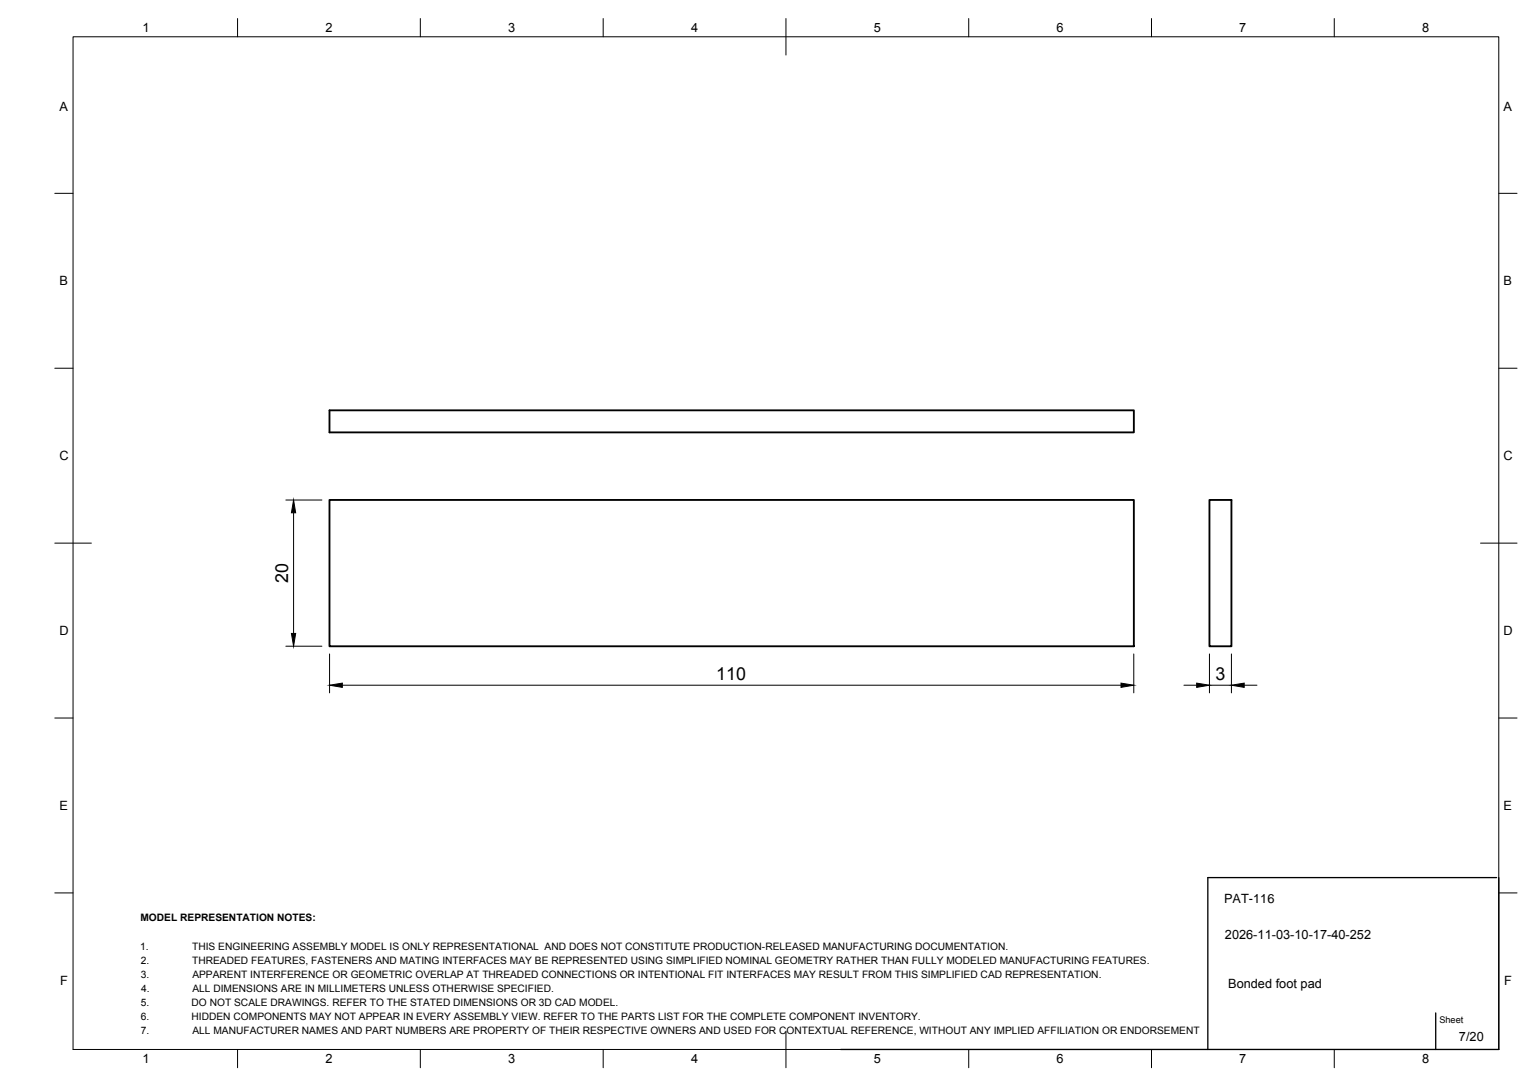
ISO-10303-21;
HEADER;
/* Generated by software containing ST-Developer
 * from STEP Tools, Inc. (www.steptools.com) 
 */

FILE_DESCRIPTION(
/* description */ ('V-block with clamp strap'),
/* implementation_level */ '2;1');

FILE_NAME(
/* name */ 'Bonded foot pad.step',
/* time_stamp */ '2026-10-27T10:50:53-07:00',
/* author */ (''),
/* organization */ (''),
/* preprocessor_version */ 'ST-DEVELOPER v20.2',
/* originating_system */ 'Autodesk Translation Framework v15.17.0.0',
/* authorisation */ '');

FILE_SCHEMA (('AUTOMOTIVE_DESIGN { 1 0 10303 214 3 1 1 }'));
ENDSEC;

DATA;
#10=MECHANICAL_DESIGN_GEOMETRIC_PRESENTATION_REPRESENTATION('',(#268),#7344);
#226=SHAPE_REPRESENTATION_RELATIONSHIP('SRR','None',#7444,#247);
#247=ADVANCED_BREP_SHAPE_REPRESENTATION('',(#289),#7323);
#268=STYLED_ITEM('',(#7624),#289);
#289=MANIFOLD_SOLID_BREP('Body1',#4150);
#598=FACE_OUTER_BOUND('',#868,.T.);
#599=FACE_OUTER_BOUND('',#869,.T.);
#600=FACE_OUTER_BOUND('',#870,.T.);
#601=FACE_OUTER_BOUND('',#871,.T.);
#602=FACE_OUTER_BOUND('',#872,.T.);
#603=FACE_OUTER_BOUND('',#873,.T.);
#868=EDGE_LOOP('',(#2876,#2877,#2878,#2879));
#869=EDGE_LOOP('',(#2880,#2881,#2882,#2883));
#870=EDGE_LOOP('',(#2884,#2885,#2886,#2887));
#871=EDGE_LOOP('',(#2888,#2889,#2890,#2891));
#872=EDGE_LOOP('',(#2892,#2893,#2894,#2895));
#873=EDGE_LOOP('',(#2896,#2897,#2898,#2899));
#1175=LINE('',#6280,#1540);
#1176=LINE('',#6282,#1541);
#1177=LINE('',#6284,#1542);
#1178=LINE('',#6285,#1543);
#1179=LINE('',#6288,#1544);
#1180=LINE('',#6290,#1545);
#1181=LINE('',#6291,#1546);
#1182=LINE('',#6294,#1547);
#1183=LINE('',#6296,#1548);
#1184=LINE('',#6297,#1549);
#1185=LINE('',#6299,#1550);
#1186=LINE('',#6300,#1551);
#1540=VECTOR('',#5045,1.);
#1541=VECTOR('',#5046,1.);
#1542=VECTOR('',#5047,1.);
#1543=VECTOR('',#5048,1.);
#1544=VECTOR('',#5051,1.);
#1545=VECTOR('',#5052,1.);
#1546=VECTOR('',#5053,1.);
#1547=VECTOR('',#5056,1.);
#1548=VECTOR('',#5057,1.);
#1549=VECTOR('',#5058,1.);
#1550=VECTOR('',#5061,1.);
#1551=VECTOR('',#5062,1.);
#1903=VERTEX_POINT('',#6278);
#1904=VERTEX_POINT('',#6279);
#1905=VERTEX_POINT('',#6281);
#1906=VERTEX_POINT('',#6283);
#1907=VERTEX_POINT('',#6287);
#1908=VERTEX_POINT('',#6289);
#1909=VERTEX_POINT('',#6293);
#1910=VERTEX_POINT('',#6295);
#2264=EDGE_CURVE('',#1903,#1904,#1175,.T.);
#2265=EDGE_CURVE('',#1904,#1905,#1176,.T.);
#2266=EDGE_CURVE('',#1906,#1905,#1177,.T.);
#2267=EDGE_CURVE('',#1903,#1906,#1178,.T.);
#2268=EDGE_CURVE('',#1907,#1903,#1179,.T.);
#2269=EDGE_CURVE('',#1908,#1906,#1180,.T.);
#2270=EDGE_CURVE('',#1907,#1908,#1181,.T.);
#2271=EDGE_CURVE('',#1909,#1907,#1182,.T.);
#2272=EDGE_CURVE('',#1910,#1908,#1183,.T.);
#2273=EDGE_CURVE('',#1909,#1910,#1184,.T.);
#2274=EDGE_CURVE('',#1904,#1909,#1185,.T.);
#2275=EDGE_CURVE('',#1905,#1910,#1186,.T.);
#2876=ORIENTED_EDGE('',*,*,#2264,.T.);
#2877=ORIENTED_EDGE('',*,*,#2265,.T.);
#2878=ORIENTED_EDGE('',*,*,#2266,.F.);
#2879=ORIENTED_EDGE('',*,*,#2267,.F.);
#2880=ORIENTED_EDGE('',*,*,#2268,.T.);
#2881=ORIENTED_EDGE('',*,*,#2267,.T.);
#2882=ORIENTED_EDGE('',*,*,#2269,.F.);
#2883=ORIENTED_EDGE('',*,*,#2270,.F.);
#2884=ORIENTED_EDGE('',*,*,#2271,.T.);
#2885=ORIENTED_EDGE('',*,*,#2270,.T.);
#2886=ORIENTED_EDGE('',*,*,#2272,.F.);
#2887=ORIENTED_EDGE('',*,*,#2273,.F.);
#2888=ORIENTED_EDGE('',*,*,#2274,.T.);
#2889=ORIENTED_EDGE('',*,*,#2273,.T.);
#2890=ORIENTED_EDGE('',*,*,#2275,.F.);
#2891=ORIENTED_EDGE('',*,*,#2265,.F.);
#2892=ORIENTED_EDGE('',*,*,#2275,.T.);
#2893=ORIENTED_EDGE('',*,*,#2272,.T.);
#2894=ORIENTED_EDGE('',*,*,#2269,.T.);
#2895=ORIENTED_EDGE('',*,*,#2266,.T.);
#2896=ORIENTED_EDGE('',*,*,#2274,.F.);
#2897=ORIENTED_EDGE('',*,*,#2264,.F.);
#2898=ORIENTED_EDGE('',*,*,#2268,.F.);
#2899=ORIENTED_EDGE('',*,*,#2271,.F.);
#3762=PLANE('',#4473);
#3763=PLANE('',#4474);
#3764=PLANE('',#4475);
#3765=PLANE('',#4476);
#3766=PLANE('',#4477);
#3767=PLANE('',#4478);
#3944=ADVANCED_FACE('',(#598),#3762,.T.);
#3945=ADVANCED_FACE('',(#599),#3763,.T.);
#3946=ADVANCED_FACE('',(#600),#3764,.T.);
#3947=ADVANCED_FACE('',(#601),#3765,.T.);
#3948=ADVANCED_FACE('',(#602),#3766,.T.);
#3949=ADVANCED_FACE('',(#603),#3767,.F.);
#4150=CLOSED_SHELL('',(#3944,#3945,#3946,#3947,#3948,#3949));
#4472=AXIS2_PLACEMENT_3D('',#6276,#5041,#5042);
#4473=AXIS2_PLACEMENT_3D('',#6277,#5043,#5044);
#4474=AXIS2_PLACEMENT_3D('',#6286,#5049,#5050);
#4475=AXIS2_PLACEMENT_3D('',#6292,#5054,#5055);
#4476=AXIS2_PLACEMENT_3D('',#6298,#5059,#5060);
#4477=AXIS2_PLACEMENT_3D('',#6301,#5063,#5064);
#4478=AXIS2_PLACEMENT_3D('',#6302,#5065,#5066);
#5041=DIRECTION('axis',(0.,0.,1.));
#5042=DIRECTION('refdir',(1.,0.,0.));
#5043=DIRECTION('center_axis',(0.,1.,0.));
#5044=DIRECTION('ref_axis',(-1.,0.,0.));
#5045=DIRECTION('',(-1.,0.,0.));
#5046=DIRECTION('',(0.,0.,1.));
#5047=DIRECTION('',(-1.,0.,0.));
#5048=DIRECTION('',(0.,0.,1.));
#5049=DIRECTION('center_axis',(1.,0.,0.));
#5050=DIRECTION('ref_axis',(0.,1.,0.));
#5051=DIRECTION('',(0.,1.,0.));
#5052=DIRECTION('',(0.,1.,0.));
#5053=DIRECTION('',(0.,0.,1.));
#5054=DIRECTION('center_axis',(0.,-1.,0.));
#5055=DIRECTION('ref_axis',(1.,0.,0.));
#5056=DIRECTION('',(1.,0.,0.));
#5057=DIRECTION('',(1.,0.,0.));
#5058=DIRECTION('',(0.,0.,1.));
#5059=DIRECTION('center_axis',(-1.,0.,0.));
#5060=DIRECTION('ref_axis',(0.,-1.,0.));
#5061=DIRECTION('',(0.,-1.,0.));
#5062=DIRECTION('',(0.,-1.,0.));
#5063=DIRECTION('center_axis',(0.,0.,1.));
#5064=DIRECTION('ref_axis',(1.,0.,0.));
#5065=DIRECTION('center_axis',(0.,0.,1.));
#5066=DIRECTION('ref_axis',(1.,0.,0.));
#6276=CARTESIAN_POINT('',(0.,0.,0.));
#6277=CARTESIAN_POINT('Origin',(4.,5.5,-1.3));
#6278=CARTESIAN_POINT('',(4.,5.5,-1.3));
#6279=CARTESIAN_POINT('',(2.,5.5,-1.3));
#6280=CARTESIAN_POINT('',(4.,5.5,-1.3));
#6281=CARTESIAN_POINT('',(2.,5.5,-1.));
#6282=CARTESIAN_POINT('',(2.,5.5,-1.3));
#6283=CARTESIAN_POINT('',(4.,5.5,-1.));
#6284=CARTESIAN_POINT('',(4.,5.5,-1.));
#6285=CARTESIAN_POINT('',(4.,5.5,-1.3));
#6286=CARTESIAN_POINT('Origin',(4.,-5.5,-1.3));
#6287=CARTESIAN_POINT('',(4.,-5.5,-1.3));
#6288=CARTESIAN_POINT('',(4.,-5.5,-1.3));
#6289=CARTESIAN_POINT('',(4.,-5.5,-1.));
#6290=CARTESIAN_POINT('',(4.,-5.5,-1.));
#6291=CARTESIAN_POINT('',(4.,-5.5,-1.3));
#6292=CARTESIAN_POINT('Origin',(2.,-5.5,-1.3));
#6293=CARTESIAN_POINT('',(2.,-5.5,-1.3));
#6294=CARTESIAN_POINT('',(2.,-5.5,-1.3));
#6295=CARTESIAN_POINT('',(2.,-5.5,-1.));
#6296=CARTESIAN_POINT('',(2.,-5.5,-1.));
#6297=CARTESIAN_POINT('',(2.,-5.5,-1.3));
#6298=CARTESIAN_POINT('Origin',(2.,5.5,-1.3));
#6299=CARTESIAN_POINT('',(2.,5.5,-1.3));
#6300=CARTESIAN_POINT('',(2.,5.5,-1.));
#6301=CARTESIAN_POINT('Origin',(3.,0.,-1.));
#6302=CARTESIAN_POINT('Origin',(3.,0.,-1.3));
#7297=UNCERTAINTY_MEASURE_WITH_UNIT(LENGTH_MEASURE(0.001),#7345,
'DISTANCE_ACCURACY_VALUE',
'Maximum model space distance between geometric entities at asserted c
onnectivities');
#7318=UNCERTAINTY_MEASURE_WITH_UNIT(LENGTH_MEASURE(0.001),#7345,
'DISTANCE_ACCURACY_VALUE',
'Maximum model space distance between geometric entities at asserted c
onnectivities');
#7323=(
GEOMETRIC_REPRESENTATION_CONTEXT(3)
GLOBAL_UNCERTAINTY_ASSIGNED_CONTEXT((#7297))
GLOBAL_UNIT_ASSIGNED_CONTEXT((#7345,#7347,#7348))
REPRESENTATION_CONTEXT('','3D')
);
#7344=(
GEOMETRIC_REPRESENTATION_CONTEXT(3)
GLOBAL_UNCERTAINTY_ASSIGNED_CONTEXT((#7318))
GLOBAL_UNIT_ASSIGNED_CONTEXT((#7345,#7347,#7348))
REPRESENTATION_CONTEXT('','3D')
);
#7345=(
LENGTH_UNIT()
NAMED_UNIT(*)
SI_UNIT(.CENTI.,.METRE.)
);
#7347=(
NAMED_UNIT(*)
PLANE_ANGLE_UNIT()
SI_UNIT($,.RADIAN.)
);
#7348=(
NAMED_UNIT(*)
SI_UNIT($,.STERADIAN.)
SOLID_ANGLE_UNIT()
);
#7353=SHAPE_DEFINITION_REPRESENTATION(#7378,#7444);
#7378=PRODUCT_DEFINITION_SHAPE('',$,#7470);
#7444=SHAPE_REPRESENTATION('',(#4472),#7323);
#7465=PRODUCT_DEFINITION_CONTEXT('part definition',#7542,'design');
#7470=PRODUCT_DEFINITION('Bonded foot pad','Bonded foot pad',#7495,#7465);
#7495=PRODUCT_DEFINITION_FORMATION('',$,#7548);
#7542=APPLICATION_CONTEXT(
'Core Data for Automotive Mechanical Design Process');
#7543=PRODUCT_CONTEXT('part definition',#7542,'mechanical');
#7548=PRODUCT('Bonded foot pad','Bonded foot pad','Bonded foot pad',(#7543));
#7618=COLOUR_RGB('Sky Blue',0.24,0.69,0.87);
#7619=FILL_AREA_STYLE_COLOUR('',#7618);
#7620=FILL_AREA_STYLE('',(#7619));
#7621=SURFACE_STYLE_FILL_AREA(#7620);
#7622=SURFACE_SIDE_STYLE('',(#7621));
#7623=SURFACE_STYLE_USAGE(.BOTH.,#7622);
#7624=PRESENTATION_STYLE_ASSIGNMENT((#7623));
ENDSEC;
END-ISO-10303-21;
